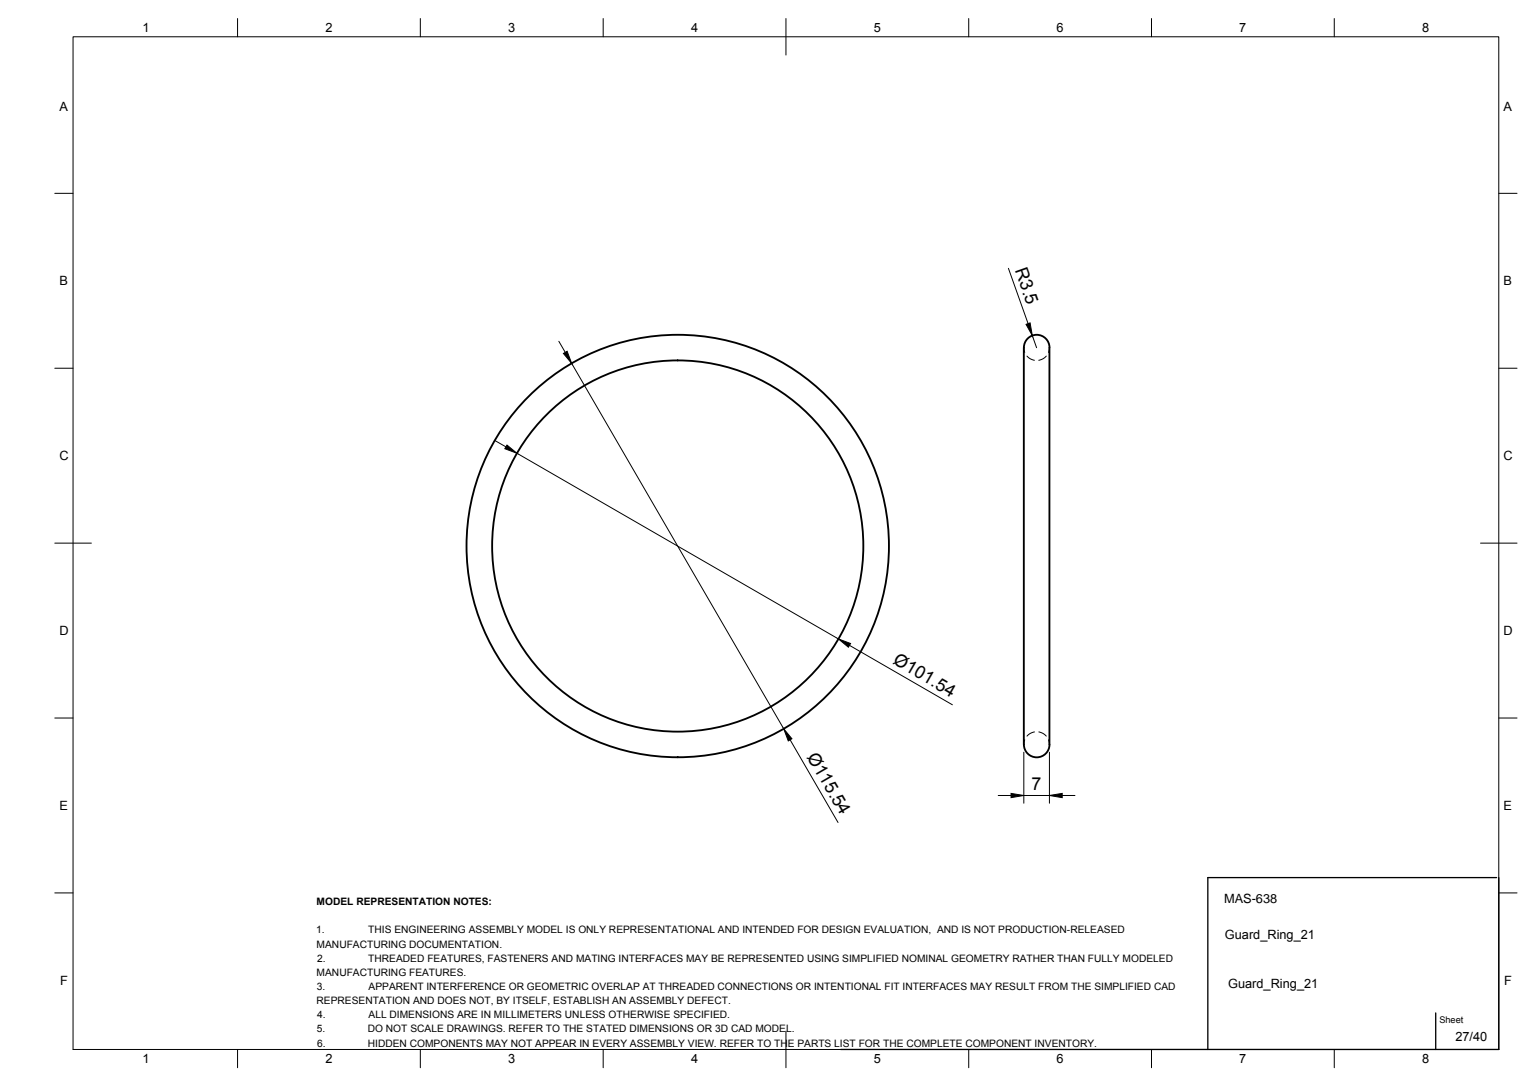
ISO-10303-21;
HEADER;
FILE_DESCRIPTION((''),'2;1');
FILE_NAME('Guard_Ring_21.step','2026-10-09T12:00:21-07:00',(''),(''),'','','');
FILE_SCHEMA (('AUTOMOTIVE_DESIGN { 1 0 10303 214 3 1 1 }'));
ENDSEC;
DATA;
#10=MECHANICAL_DESIGN_GEOMETRIC_PRESENTATION_REPRESENTATION('',(#426),#10334);
#354=SHAPE_REPRESENTATION_RELATIONSHIP('SRR','None',#10470,#386) ;
#386=ADVANCED_BREP_SHAPE_REPRESENTATION('',(#458),#10322) ;
#426=STYLED_ITEM('',(#10632),#458) ;
#458=MANIFOLD_SOLID_BREP('Body1',#3580) ;
#879=FACE_OUTER_BOUND('',#1079,.T.) ;
#1079=EDGE_LOOP('',(#2429,#2430,#2431,#2432)) ;
#1316=CIRCLE('',#4055,0.349999999999999) ;
#1317=CIRCLE('',#4056,5.07681446136678) ;
#1533=VERTEX_POINT('',#5753) ;
#1871=EDGE_CURVE('',#1533,#1533,#1316,.T.) ;
#1872=EDGE_CURVE('',#1533,#1533,#1317,.T.) ;
#2429=ORIENTED_EDGE('',*,*,#1871,.F.) ;
#2430=ORIENTED_EDGE('',*,*,#1872,.T.) ;
#2431=ORIENTED_EDGE('',*,*,#1871,.T.) ;
#2432=ORIENTED_EDGE('',*,*,#1872,.F.) ;
#3325=TOROIDAL_SURFACE('',#4054,5.42681446136678,0.349999999999999) ;
#3387=ADVANCED_FACE('',(#879),#3325,.T.) ;
#3580=CLOSED_SHELL('',(#3387)) ;
#4053=AXIS2_PLACEMENT_3D('',#5751,#4667,#4668) ;
#4054=AXIS2_PLACEMENT_3D('',#5752,#4669,#4670) ;
#4055=AXIS2_PLACEMENT_3D('',#5754,#4671,#4672) ;
#4056=AXIS2_PLACEMENT_3D('',#5755,#4673,#4674) ;
#4667=DIRECTION('axis',(0.,0.,1.)) ;
#4668=DIRECTION('refdir',(1.,0.,0.)) ;
#4669=DIRECTION('center_axis',(-6.42891162084177E-17,-1.,-1.01883556321148E-16)) ;
#4670=DIRECTION('ref_axis',(1.,0.,0.)) ;
#4671=DIRECTION('center_axis',(0.,1.01883556321148E-16,-1.)) ;
#4672=DIRECTION('ref_axis',(-1.,0.,0.)) ;
#4673=DIRECTION('center_axis',(6.42891162084177E-17,1.,1.01883556321148E-16)) ;
#4674=DIRECTION('ref_axis',(1.,-6.42891162084177E-17,-6.55000379205715E-33)) ;
#5751=CARTESIAN_POINT('',(0.,0.,0.)) ;
#5752=CARTESIAN_POINT('Origin',(23.47768801576,63.1831179463143,68.2224337400009)) ;
#5753=CARTESIAN_POINT('',(18.4008735543932,63.1831179463143,68.2224337400009)) ;
#5754=CARTESIAN_POINT('Origin',(18.0508735543932,63.1831179463143,68.2224337400009)) ;
#5755=CARTESIAN_POINT('Origin',(23.47768801576,63.1831179463143,68.2224337400009)) ;
#10285=UNCERTAINTY_MEASURE_WITH_UNIT(LENGTH_MEASURE(0.001),#10335,
'DISTANCE_ACCURACY_VALUE',
'Maximum model space distance between geometric entities at asserted c
onnectivities') ;
#10297=UNCERTAINTY_MEASURE_WITH_UNIT(LENGTH_MEASURE(0.001),#10335,
'DISTANCE_ACCURACY_VALUE',
'Maximum model space distance between geometric entities at asserted c
onnectivities') ;
#10322=(
GEOMETRIC_REPRESENTATION_CONTEXT(3)
GLOBAL_UNCERTAINTY_ASSIGNED_CONTEXT((#10285))
GLOBAL_UNIT_ASSIGNED_CONTEXT((#10335,#10337,#10338))
REPRESENTATION_CONTEXT('','3D')
) ;
#10334=(
GEOMETRIC_REPRESENTATION_CONTEXT(3)
GLOBAL_UNCERTAINTY_ASSIGNED_CONTEXT((#10297))
GLOBAL_UNIT_ASSIGNED_CONTEXT((#10335,#10337,#10338))
REPRESENTATION_CONTEXT('','3D')
) ;
#10335=(
LENGTH_UNIT()
NAMED_UNIT(*)
SI_UNIT(.CENTI.,.METRE.)
) ;
#10337=(
NAMED_UNIT(*)
PLANE_ANGLE_UNIT()
SI_UNIT($,.RADIAN.)
) ;
#10338=(
NAMED_UNIT(*)
SI_UNIT($,.STERADIAN.)
SOLID_ANGLE_UNIT()
) ;
#10363=SHAPE_DEFINITION_REPRESENTATION(#10399,#10470) ;
#10399=PRODUCT_DEFINITION_SHAPE('',$,#10507) ;
#10470=SHAPE_REPRESENTATION('',(#4053),#10322) ;
#10482=PRODUCT_DEFINITION_CONTEXT('part definition',#10592,'design') ;
#10507=PRODUCT_DEFINITION('Guard_Ring_21','Guard_Ring_21',#10543,#10482) ;
#10543=PRODUCT_DEFINITION_FORMATION('',$,#10618) ;
#10592=APPLICATION_CONTEXT(
'Core Data for Automotive Mechanical Design Process') ;
#10593=PRODUCT_CONTEXT('part definition',#10592,'mechanical') ;
#10618=PRODUCT('Guard_Ring_21','Guard_Ring_21',$,(#10593)) ;
#10632=PRESENTATION_STYLE_ASSIGNMENT((#10636)) ;
#10636=SURFACE_STYLE_USAGE(.BOTH.,#10640) ;
#10640=SURFACE_SIDE_STYLE('',(#10644)) ;
#10644=SURFACE_STYLE_FILL_AREA(#10648) ;
#10648=FILL_AREA_STYLE('Opaque(202,209,238)',(#10652)) ;
#10652=FILL_AREA_STYLE_COLOUR('Opaque(202,209,238)',#10656) ;
#10656=COLOUR_RGB('Opaque(202,209,238)', 0.40784314, 0.44705882, 0.49803922) ;
ENDSEC;
END-ISO-10303-21;
